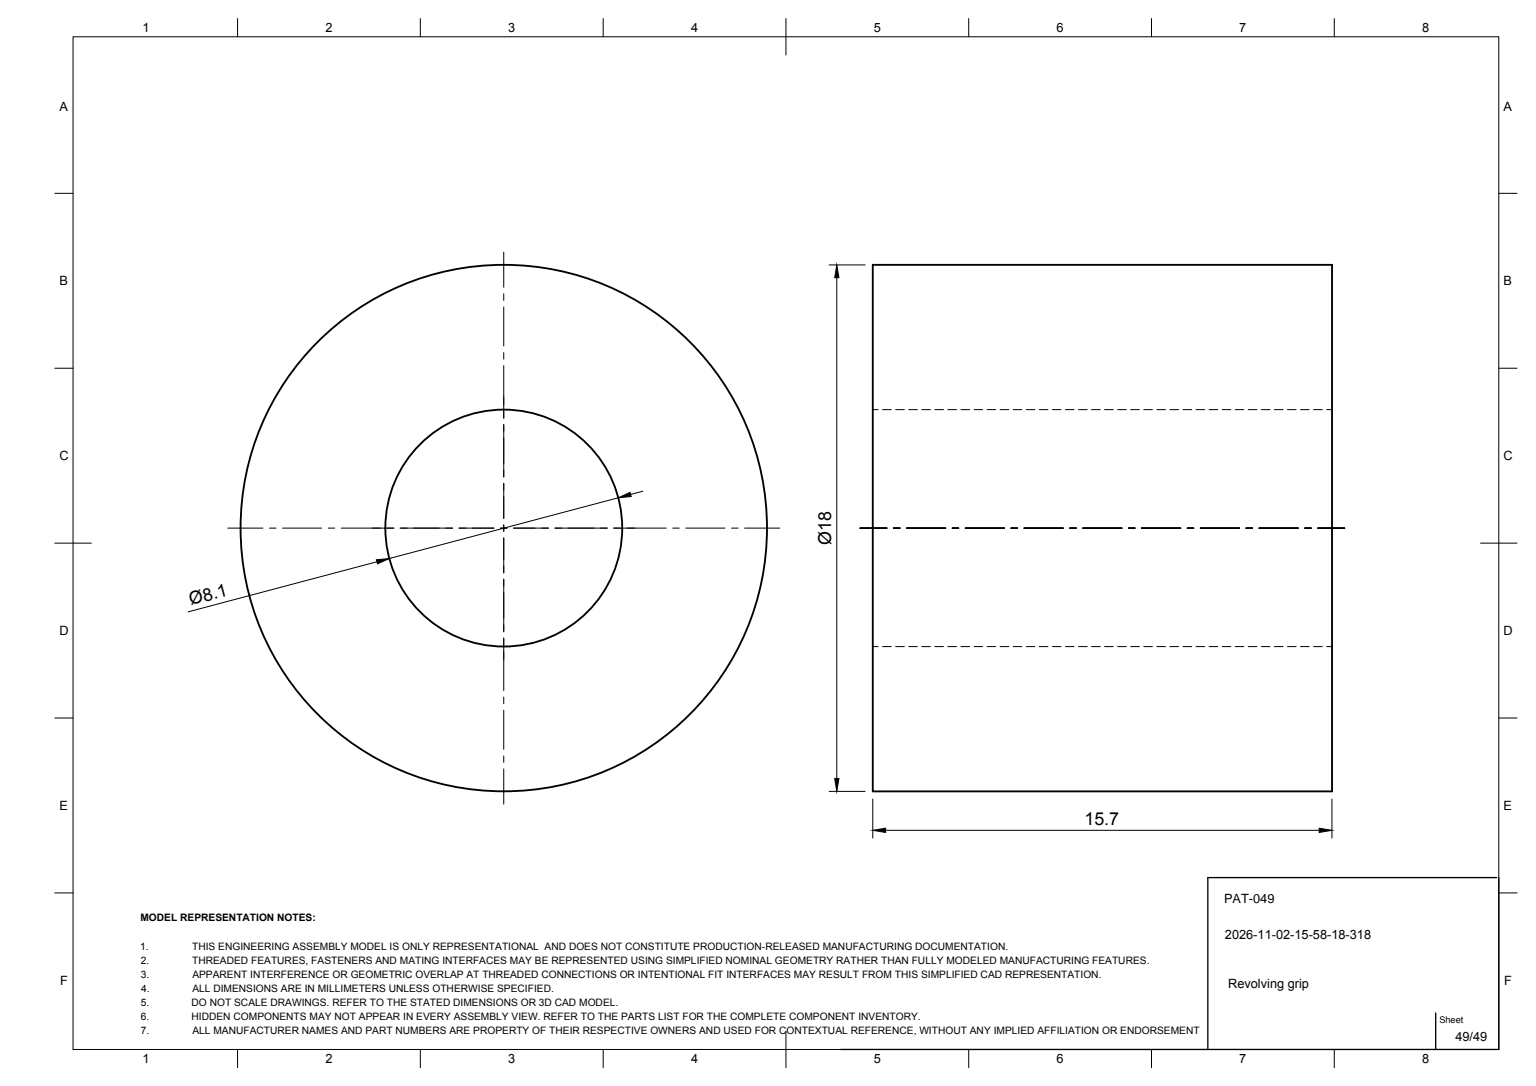
ISO-10303-21;
HEADER;
/* Generated by software containing ST-Developer
 * from STEP Tools, Inc. (www.steptools.com) 
 */

FILE_DESCRIPTION(
/* description */ ('Hand drill press frame (manual)'),
/* implementation_level */ '2;1');

FILE_NAME(
/* name */ 'Revolving grip.step',
/* time_stamp */ '2026-10-28T03:25:28-07:00',
/* author */ (''),
/* organization */ (''),
/* preprocessor_version */ 'ST-DEVELOPER v20.2',
/* originating_system */ 'Autodesk Translation Framework v15.17.0.0',
/* authorisation */ '');

FILE_SCHEMA (('AUTOMOTIVE_DESIGN { 1 0 10303 214 3 1 1 }'));
ENDSEC;

DATA;
#10=MECHANICAL_DESIGN_GEOMETRIC_PRESENTATION_REPRESENTATION('',(#670),#33299);
#573=SHAPE_REPRESENTATION_RELATIONSHIP('SRR','None',#33536,#618);
#618=ADVANCED_BREP_SHAPE_REPRESENTATION('',(#719),#33298);
#670=STYLED_ITEM('',(#33821),#719);
#719=MANIFOLD_SOLID_BREP('Body1',#12691);
#885=FACE_BOUND('',#2881,.T.);
#886=FACE_BOUND('',#2883,.T.);
#1337=PLANE('',#14360);
#1338=PLANE('',#14361);
#2024=FACE_OUTER_BOUND('',#2878,.T.);
#2025=FACE_OUTER_BOUND('',#2879,.T.);
#2026=FACE_OUTER_BOUND('',#2880,.T.);
#2027=FACE_OUTER_BOUND('',#2882,.T.);
#2878=EDGE_LOOP('',(#11773,#11774,#11775,#11776));
#2879=EDGE_LOOP('',(#11777,#11778,#11779,#11780));
#2880=EDGE_LOOP('',(#11781));
#2881=EDGE_LOOP('',(#11782));
#2882=EDGE_LOOP('',(#11783));
#2883=EDGE_LOOP('',(#11784));
#4047=LINE('',#33181,#5212);
#4048=LINE('',#33187,#5213);
#5212=VECTOR('',#17866,0.405);
#5213=VECTOR('',#17873,0.9);
#5609=CIRCLE('',#14355,0.405);
#5610=CIRCLE('',#14356,0.405);
#5611=CIRCLE('',#14358,0.9);
#5612=CIRCLE('',#14359,0.9);
#6735=VERTEX_POINT('',#33178);
#6736=VERTEX_POINT('',#33180);
#6737=VERTEX_POINT('',#33184);
#6738=VERTEX_POINT('',#33186);
#8415=EDGE_CURVE('',#6735,#6735,#5609,.T.);
#8416=EDGE_CURVE('',#6735,#6736,#4047,.T.);
#8417=EDGE_CURVE('',#6736,#6736,#5610,.T.);
#8418=EDGE_CURVE('',#6737,#6737,#5611,.T.);
#8419=EDGE_CURVE('',#6737,#6738,#4048,.T.);
#8420=EDGE_CURVE('',#6738,#6738,#5612,.T.);
#11773=ORIENTED_EDGE('',*,*,#8415,.F.);
#11774=ORIENTED_EDGE('',*,*,#8416,.T.);
#11775=ORIENTED_EDGE('',*,*,#8417,.T.);
#11776=ORIENTED_EDGE('',*,*,#8416,.F.);
#11777=ORIENTED_EDGE('',*,*,#8418,.F.);
#11778=ORIENTED_EDGE('',*,*,#8419,.T.);
#11779=ORIENTED_EDGE('',*,*,#8420,.T.);
#11780=ORIENTED_EDGE('',*,*,#8419,.F.);
#11781=ORIENTED_EDGE('',*,*,#8418,.T.);
#11782=ORIENTED_EDGE('',*,*,#8415,.T.);
#11783=ORIENTED_EDGE('',*,*,#8420,.F.);
#11784=ORIENTED_EDGE('',*,*,#8417,.F.);
#11946=CYLINDRICAL_SURFACE('',#14354,0.405);
#11947=CYLINDRICAL_SURFACE('',#14357,0.9);
#12633=ADVANCED_FACE('',(#2024),#11946,.F.);
#12634=ADVANCED_FACE('',(#2025),#11947,.T.);
#12635=ADVANCED_FACE('',(#2026,#885),#1337,.T.);
#12636=ADVANCED_FACE('',(#2027,#886),#1338,.F.);
#12691=CLOSED_SHELL('',(#12633,#12634,#12635,#12636));
#14353=AXIS2_PLACEMENT_3D('',#33176,#17860,#17861);
#14354=AXIS2_PLACEMENT_3D('',#33177,#17862,#17863);
#14355=AXIS2_PLACEMENT_3D('',#33179,#17864,#17865);
#14356=AXIS2_PLACEMENT_3D('',#33182,#17867,#17868);
#14357=AXIS2_PLACEMENT_3D('',#33183,#17869,#17870);
#14358=AXIS2_PLACEMENT_3D('',#33185,#17871,#17872);
#14359=AXIS2_PLACEMENT_3D('',#33188,#17874,#17875);
#14360=AXIS2_PLACEMENT_3D('',#33189,#17876,#17877);
#14361=AXIS2_PLACEMENT_3D('',#33190,#17878,#17879);
#17860=DIRECTION('axis',(0.,0.,1.));
#17861=DIRECTION('refdir',(1.,0.,0.));
#17862=DIRECTION('center_axis',(0.,1.,0.));
#17863=DIRECTION('ref_axis',(1.,0.,0.));
#17864=DIRECTION('center_axis',(0.,-1.,0.));
#17865=DIRECTION('ref_axis',(1.,0.,0.));
#17866=DIRECTION('',(0.,-1.,0.));
#17867=DIRECTION('center_axis',(0.,-1.,0.));
#17868=DIRECTION('ref_axis',(1.,0.,0.));
#17869=DIRECTION('center_axis',(0.,1.,0.));
#17870=DIRECTION('ref_axis',(1.,0.,0.));
#17871=DIRECTION('center_axis',(0.,1.,0.));
#17872=DIRECTION('ref_axis',(1.,0.,0.));
#17873=DIRECTION('',(0.,-1.,0.));
#17874=DIRECTION('center_axis',(0.,1.,0.));
#17875=DIRECTION('ref_axis',(1.,0.,0.));
#17876=DIRECTION('center_axis',(0.,1.,0.));
#17877=DIRECTION('ref_axis',(1.,0.,0.));
#17878=DIRECTION('center_axis',(0.,1.,0.));
#17879=DIRECTION('ref_axis',(1.,0.,0.));
#33176=CARTESIAN_POINT('',(0.,0.,0.));
#33177=CARTESIAN_POINT('Origin',(-3.25,6.8,29.));
#33178=CARTESIAN_POINT('',(-3.655,8.37,29.));
#33179=CARTESIAN_POINT('Origin',(-3.25,8.37,29.));
#33180=CARTESIAN_POINT('',(-3.655,6.8,29.));
#33181=CARTESIAN_POINT('',(-3.655,6.8,29.));
#33182=CARTESIAN_POINT('Origin',(-3.25,6.8,29.));
#33183=CARTESIAN_POINT('Origin',(-3.25,6.8,29.));
#33184=CARTESIAN_POINT('',(-4.15,8.37,29.));
#33185=CARTESIAN_POINT('Origin',(-3.25,8.37,29.));
#33186=CARTESIAN_POINT('',(-4.15,6.8,29.));
#33187=CARTESIAN_POINT('',(-4.15,6.8,29.));
#33188=CARTESIAN_POINT('Origin',(-3.25,6.8,29.));
#33189=CARTESIAN_POINT('Origin',(-3.25,8.37,29.));
#33190=CARTESIAN_POINT('Origin',(-3.25,6.8,29.));
#33246=UNCERTAINTY_MEASURE_WITH_UNIT(LENGTH_MEASURE(0.001),#33300,
'DISTANCE_ACCURACY_VALUE',
'Maximum model space distance between geometric entities at asserted c
onnectivities');
#33247=UNCERTAINTY_MEASURE_WITH_UNIT(LENGTH_MEASURE(0.001),#33300,
'DISTANCE_ACCURACY_VALUE',
'Maximum model space distance between geometric entities at asserted c
onnectivities');
#33298=(
GEOMETRIC_REPRESENTATION_CONTEXT(3)
GLOBAL_UNCERTAINTY_ASSIGNED_CONTEXT((#33246))
GLOBAL_UNIT_ASSIGNED_CONTEXT((#33300,#33302,#33303))
REPRESENTATION_CONTEXT('','3D')
);
#33299=(
GEOMETRIC_REPRESENTATION_CONTEXT(3)
GLOBAL_UNCERTAINTY_ASSIGNED_CONTEXT((#33247))
GLOBAL_UNIT_ASSIGNED_CONTEXT((#33300,#33302,#33303))
REPRESENTATION_CONTEXT('','3D')
);
#33300=(
LENGTH_UNIT()
NAMED_UNIT(*)
SI_UNIT(.CENTI.,.METRE.)
);
#33302=(
NAMED_UNIT(*)
PLANE_ANGLE_UNIT()
SI_UNIT($,.RADIAN.)
);
#33303=(
NAMED_UNIT(*)
SI_UNIT($,.STERADIAN.)
SOLID_ANGLE_UNIT()
);
#33354=SHAPE_DEFINITION_REPRESENTATION(#33480,#33536);
#33480=PRODUCT_DEFINITION_SHAPE('',$,#33588);
#33536=SHAPE_REPRESENTATION('',(#14353),#33298);
#33537=PRODUCT_DEFINITION_CONTEXT('part definition',#33692,'design');
#33588=PRODUCT_DEFINITION('Revolving grip','Revolving grip',#33639,#33537);
#33639=PRODUCT_DEFINITION_FORMATION('',$,#33744);
#33692=APPLICATION_CONTEXT(
'Core Data for Automotive Mechanical Design Process');
#33693=PRODUCT_CONTEXT('part definition',#33692,'mechanical');
#33744=PRODUCT('Revolving grip','Revolving grip','Revolving grip',(#33693));
#33815=COLOUR_RGB('Black',0.12,0.14,0.17);
#33816=FILL_AREA_STYLE_COLOUR('',#33815);
#33817=FILL_AREA_STYLE('',(#33816));
#33818=SURFACE_STYLE_FILL_AREA(#33817);
#33819=SURFACE_SIDE_STYLE('',(#33818));
#33820=SURFACE_STYLE_USAGE(.BOTH.,#33819);
#33821=PRESENTATION_STYLE_ASSIGNMENT((#33820));
ENDSEC;
END-ISO-10303-21;
